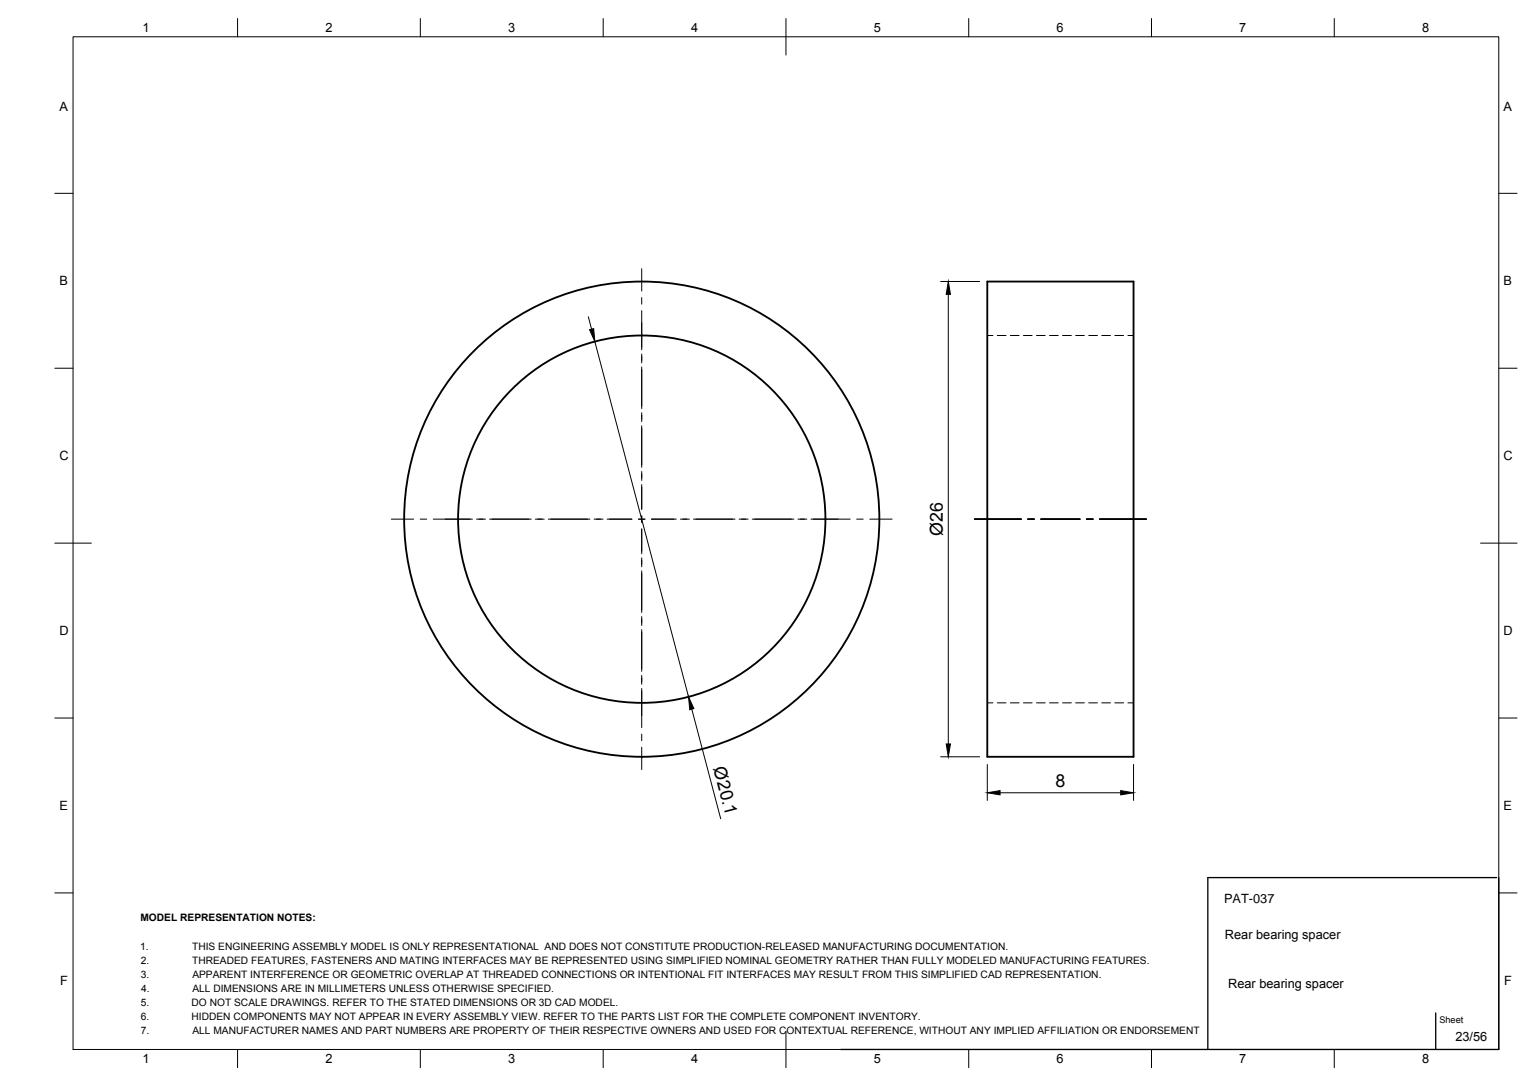
ISO-10303-21;
HEADER;
/* Generated by software containing ST-Developer
 * from STEP Tools, Inc. (www.steptools.com) 
 */

FILE_DESCRIPTION(
/* description */ ('Flywheel Crank-Slider'),
/* implementation_level */ '2;1');

FILE_NAME(
/* name */ 'Rear bearing spacer.step',
/* time_stamp */ '2026-10-28T03:23:13-07:00',
/* author */ (''),
/* organization */ (''),
/* preprocessor_version */ 'ST-DEVELOPER v20.2',
/* originating_system */ 'Autodesk Translation Framework v15.17.0.0',
/* authorisation */ '');

FILE_SCHEMA (('AUTOMOTIVE_DESIGN { 1 0 10303 214 3 1 1 }'));
ENDSEC;

DATA;
#10=MECHANICAL_DESIGN_GEOMETRIC_PRESENTATION_REPRESENTATION('',(#693),#17322);
#588=SHAPE_REPRESENTATION_RELATIONSHIP('SRR','None',#17586,#640);
#640=ADVANCED_BREP_SHAPE_REPRESENTATION('',(#750),#17290);
#693=STYLED_ITEM('',(#17931),#750);
#750=MANIFOLD_SOLID_BREP('Body1',#9075);
#916=FACE_BOUND('',#2285,.T.);
#917=FACE_BOUND('',#2287,.T.);
#1189=PLANE('',#10234);
#1190=PLANE('',#10235);
#1616=FACE_OUTER_BOUND('',#2282,.T.);
#1617=FACE_OUTER_BOUND('',#2283,.T.);
#1618=FACE_OUTER_BOUND('',#2284,.T.);
#1619=FACE_OUTER_BOUND('',#2286,.T.);
#2282=EDGE_LOOP('',(#7372,#7373,#7374,#7375));
#2283=EDGE_LOOP('',(#7376,#7377,#7378,#7379));
#2284=EDGE_LOOP('',(#7380));
#2285=EDGE_LOOP('',(#7381));
#2286=EDGE_LOOP('',(#7382));
#2287=EDGE_LOOP('',(#7383));
#2993=LINE('',#15629,#3604);
#2994=LINE('',#15635,#3605);
#3604=VECTOR('',#12297,1.005);
#3605=VECTOR('',#12304,1.3);
#4054=CIRCLE('',#10229,1.005);
#4055=CIRCLE('',#10230,1.005);
#4056=CIRCLE('',#10232,1.3);
#4057=CIRCLE('',#10233,1.3);
#4691=VERTEX_POINT('',#15626);
#4692=VERTEX_POINT('',#15628);
#4693=VERTEX_POINT('',#15632);
#4694=VERTEX_POINT('',#15634);
#5643=EDGE_CURVE('',#4691,#4691,#4054,.T.);
#5644=EDGE_CURVE('',#4691,#4692,#2993,.T.);
#5645=EDGE_CURVE('',#4692,#4692,#4055,.T.);
#5646=EDGE_CURVE('',#4693,#4693,#4056,.T.);
#5647=EDGE_CURVE('',#4693,#4694,#2994,.T.);
#5648=EDGE_CURVE('',#4694,#4694,#4057,.T.);
#7372=ORIENTED_EDGE('',*,*,#5643,.F.);
#7373=ORIENTED_EDGE('',*,*,#5644,.T.);
#7374=ORIENTED_EDGE('',*,*,#5645,.T.);
#7375=ORIENTED_EDGE('',*,*,#5644,.F.);
#7376=ORIENTED_EDGE('',*,*,#5646,.F.);
#7377=ORIENTED_EDGE('',*,*,#5647,.T.);
#7378=ORIENTED_EDGE('',*,*,#5648,.T.);
#7379=ORIENTED_EDGE('',*,*,#5647,.F.);
#7380=ORIENTED_EDGE('',*,*,#5646,.T.);
#7381=ORIENTED_EDGE('',*,*,#5643,.T.);
#7382=ORIENTED_EDGE('',*,*,#5648,.F.);
#7383=ORIENTED_EDGE('',*,*,#5645,.F.);
#8430=CYLINDRICAL_SURFACE('',#10228,1.005);
#8431=CYLINDRICAL_SURFACE('',#10231,1.3);
#8807=ADVANCED_FACE('',(#1616),#8430,.F.);
#8808=ADVANCED_FACE('',(#1617),#8431,.T.);
#8809=ADVANCED_FACE('',(#1618,#916),#1189,.T.);
#8810=ADVANCED_FACE('',(#1619,#917),#1190,.F.);
#9075=CLOSED_SHELL('',(#8807,#8808,#8809,#8810));
#10227=AXIS2_PLACEMENT_3D('',#15624,#12291,#12292);
#10228=AXIS2_PLACEMENT_3D('',#15625,#12293,#12294);
#10229=AXIS2_PLACEMENT_3D('',#15627,#12295,#12296);
#10230=AXIS2_PLACEMENT_3D('',#15630,#12298,#12299);
#10231=AXIS2_PLACEMENT_3D('',#15631,#12300,#12301);
#10232=AXIS2_PLACEMENT_3D('',#15633,#12302,#12303);
#10233=AXIS2_PLACEMENT_3D('',#15636,#12305,#12306);
#10234=AXIS2_PLACEMENT_3D('',#15637,#12307,#12308);
#10235=AXIS2_PLACEMENT_3D('',#15638,#12309,#12310);
#12291=DIRECTION('axis',(0.,0.,1.));
#12292=DIRECTION('refdir',(1.,0.,0.));
#12293=DIRECTION('center_axis',(0.,1.,0.));
#12294=DIRECTION('ref_axis',(1.,0.,0.));
#12295=DIRECTION('center_axis',(0.,-1.,0.));
#12296=DIRECTION('ref_axis',(1.,0.,0.));
#12297=DIRECTION('',(0.,-1.,0.));
#12298=DIRECTION('center_axis',(0.,-1.,0.));
#12299=DIRECTION('ref_axis',(1.,0.,0.));
#12300=DIRECTION('center_axis',(0.,1.,0.));
#12301=DIRECTION('ref_axis',(1.,0.,0.));
#12302=DIRECTION('center_axis',(0.,1.,0.));
#12303=DIRECTION('ref_axis',(1.,0.,0.));
#12304=DIRECTION('',(0.,-1.,0.));
#12305=DIRECTION('center_axis',(0.,1.,0.));
#12306=DIRECTION('ref_axis',(1.,0.,0.));
#12307=DIRECTION('center_axis',(0.,1.,0.));
#12308=DIRECTION('ref_axis',(1.,0.,0.));
#12309=DIRECTION('center_axis',(0.,1.,0.));
#12310=DIRECTION('ref_axis',(1.,0.,0.));
#15624=CARTESIAN_POINT('',(0.,0.,0.));
#15625=CARTESIAN_POINT('Origin',(0.,-16.65,10.));
#15626=CARTESIAN_POINT('',(-1.005,-15.85,10.));
#15627=CARTESIAN_POINT('Origin',(0.,-15.85,10.));
#15628=CARTESIAN_POINT('',(-1.005,-16.65,10.));
#15629=CARTESIAN_POINT('',(-1.005,-16.65,10.));
#15630=CARTESIAN_POINT('Origin',(0.,-16.65,10.));
#15631=CARTESIAN_POINT('Origin',(0.,-16.65,10.));
#15632=CARTESIAN_POINT('',(-1.3,-15.85,10.));
#15633=CARTESIAN_POINT('Origin',(0.,-15.85,10.));
#15634=CARTESIAN_POINT('',(-1.3,-16.65,10.));
#15635=CARTESIAN_POINT('',(-1.3,-16.65,10.));
#15636=CARTESIAN_POINT('Origin',(0.,-16.65,10.));
#15637=CARTESIAN_POINT('Origin',(0.,-15.85,10.));
#15638=CARTESIAN_POINT('Origin',(0.,-16.65,10.));
#17229=UNCERTAINTY_MEASURE_WITH_UNIT(LENGTH_MEASURE(0.001),#17323,
'DISTANCE_ACCURACY_VALUE',
'Maximum model space distance between geometric entities at asserted c
onnectivities');
#17261=UNCERTAINTY_MEASURE_WITH_UNIT(LENGTH_MEASURE(0.001),#17323,
'DISTANCE_ACCURACY_VALUE',
'Maximum model space distance between geometric entities at asserted c
onnectivities');
#17290=(
GEOMETRIC_REPRESENTATION_CONTEXT(3)
GLOBAL_UNCERTAINTY_ASSIGNED_CONTEXT((#17229))
GLOBAL_UNIT_ASSIGNED_CONTEXT((#17323,#17325,#17326))
REPRESENTATION_CONTEXT('','3D')
);
#17322=(
GEOMETRIC_REPRESENTATION_CONTEXT(3)
GLOBAL_UNCERTAINTY_ASSIGNED_CONTEXT((#17261))
GLOBAL_UNIT_ASSIGNED_CONTEXT((#17323,#17325,#17326))
REPRESENTATION_CONTEXT('','3D')
);
#17323=(
LENGTH_UNIT()
NAMED_UNIT(*)
SI_UNIT(.CENTI.,.METRE.)
);
#17325=(
NAMED_UNIT(*)
PLANE_ANGLE_UNIT()
SI_UNIT($,.RADIAN.)
);
#17326=(
NAMED_UNIT(*)
SI_UNIT($,.STERADIAN.)
SOLID_ANGLE_UNIT()
);
#17355=SHAPE_DEFINITION_REPRESENTATION(#17417,#17586);
#17417=PRODUCT_DEFINITION_SHAPE('',$,#17647);
#17586=SHAPE_REPRESENTATION('',(#10227),#17290);
#17618=PRODUCT_DEFINITION_CONTEXT('part definition',#17800,'design');
#17647=PRODUCT_DEFINITION('Rear bearing spacer','Rear bearing spacer',#17707,
#17618);
#17707=PRODUCT_DEFINITION_FORMATION('',$,#17830);
#17800=APPLICATION_CONTEXT(
'Core Data for Automotive Mechanical Design Process');
#17801=PRODUCT_CONTEXT('part definition',#17800,'mechanical');
#17830=PRODUCT('Rear bearing spacer','Rear bearing spacer',
'Rear bearing spacer',(#17801));
#17925=COLOUR_RGB('Grey',0.48,0.52,0.57);
#17926=FILL_AREA_STYLE_COLOUR('',#17925);
#17927=FILL_AREA_STYLE('',(#17926));
#17928=SURFACE_STYLE_FILL_AREA(#17927);
#17929=SURFACE_SIDE_STYLE('',(#17928));
#17930=SURFACE_STYLE_USAGE(.BOTH.,#17929);
#17931=PRESENTATION_STYLE_ASSIGNMENT((#17930));
ENDSEC;
END-ISO-10303-21;
